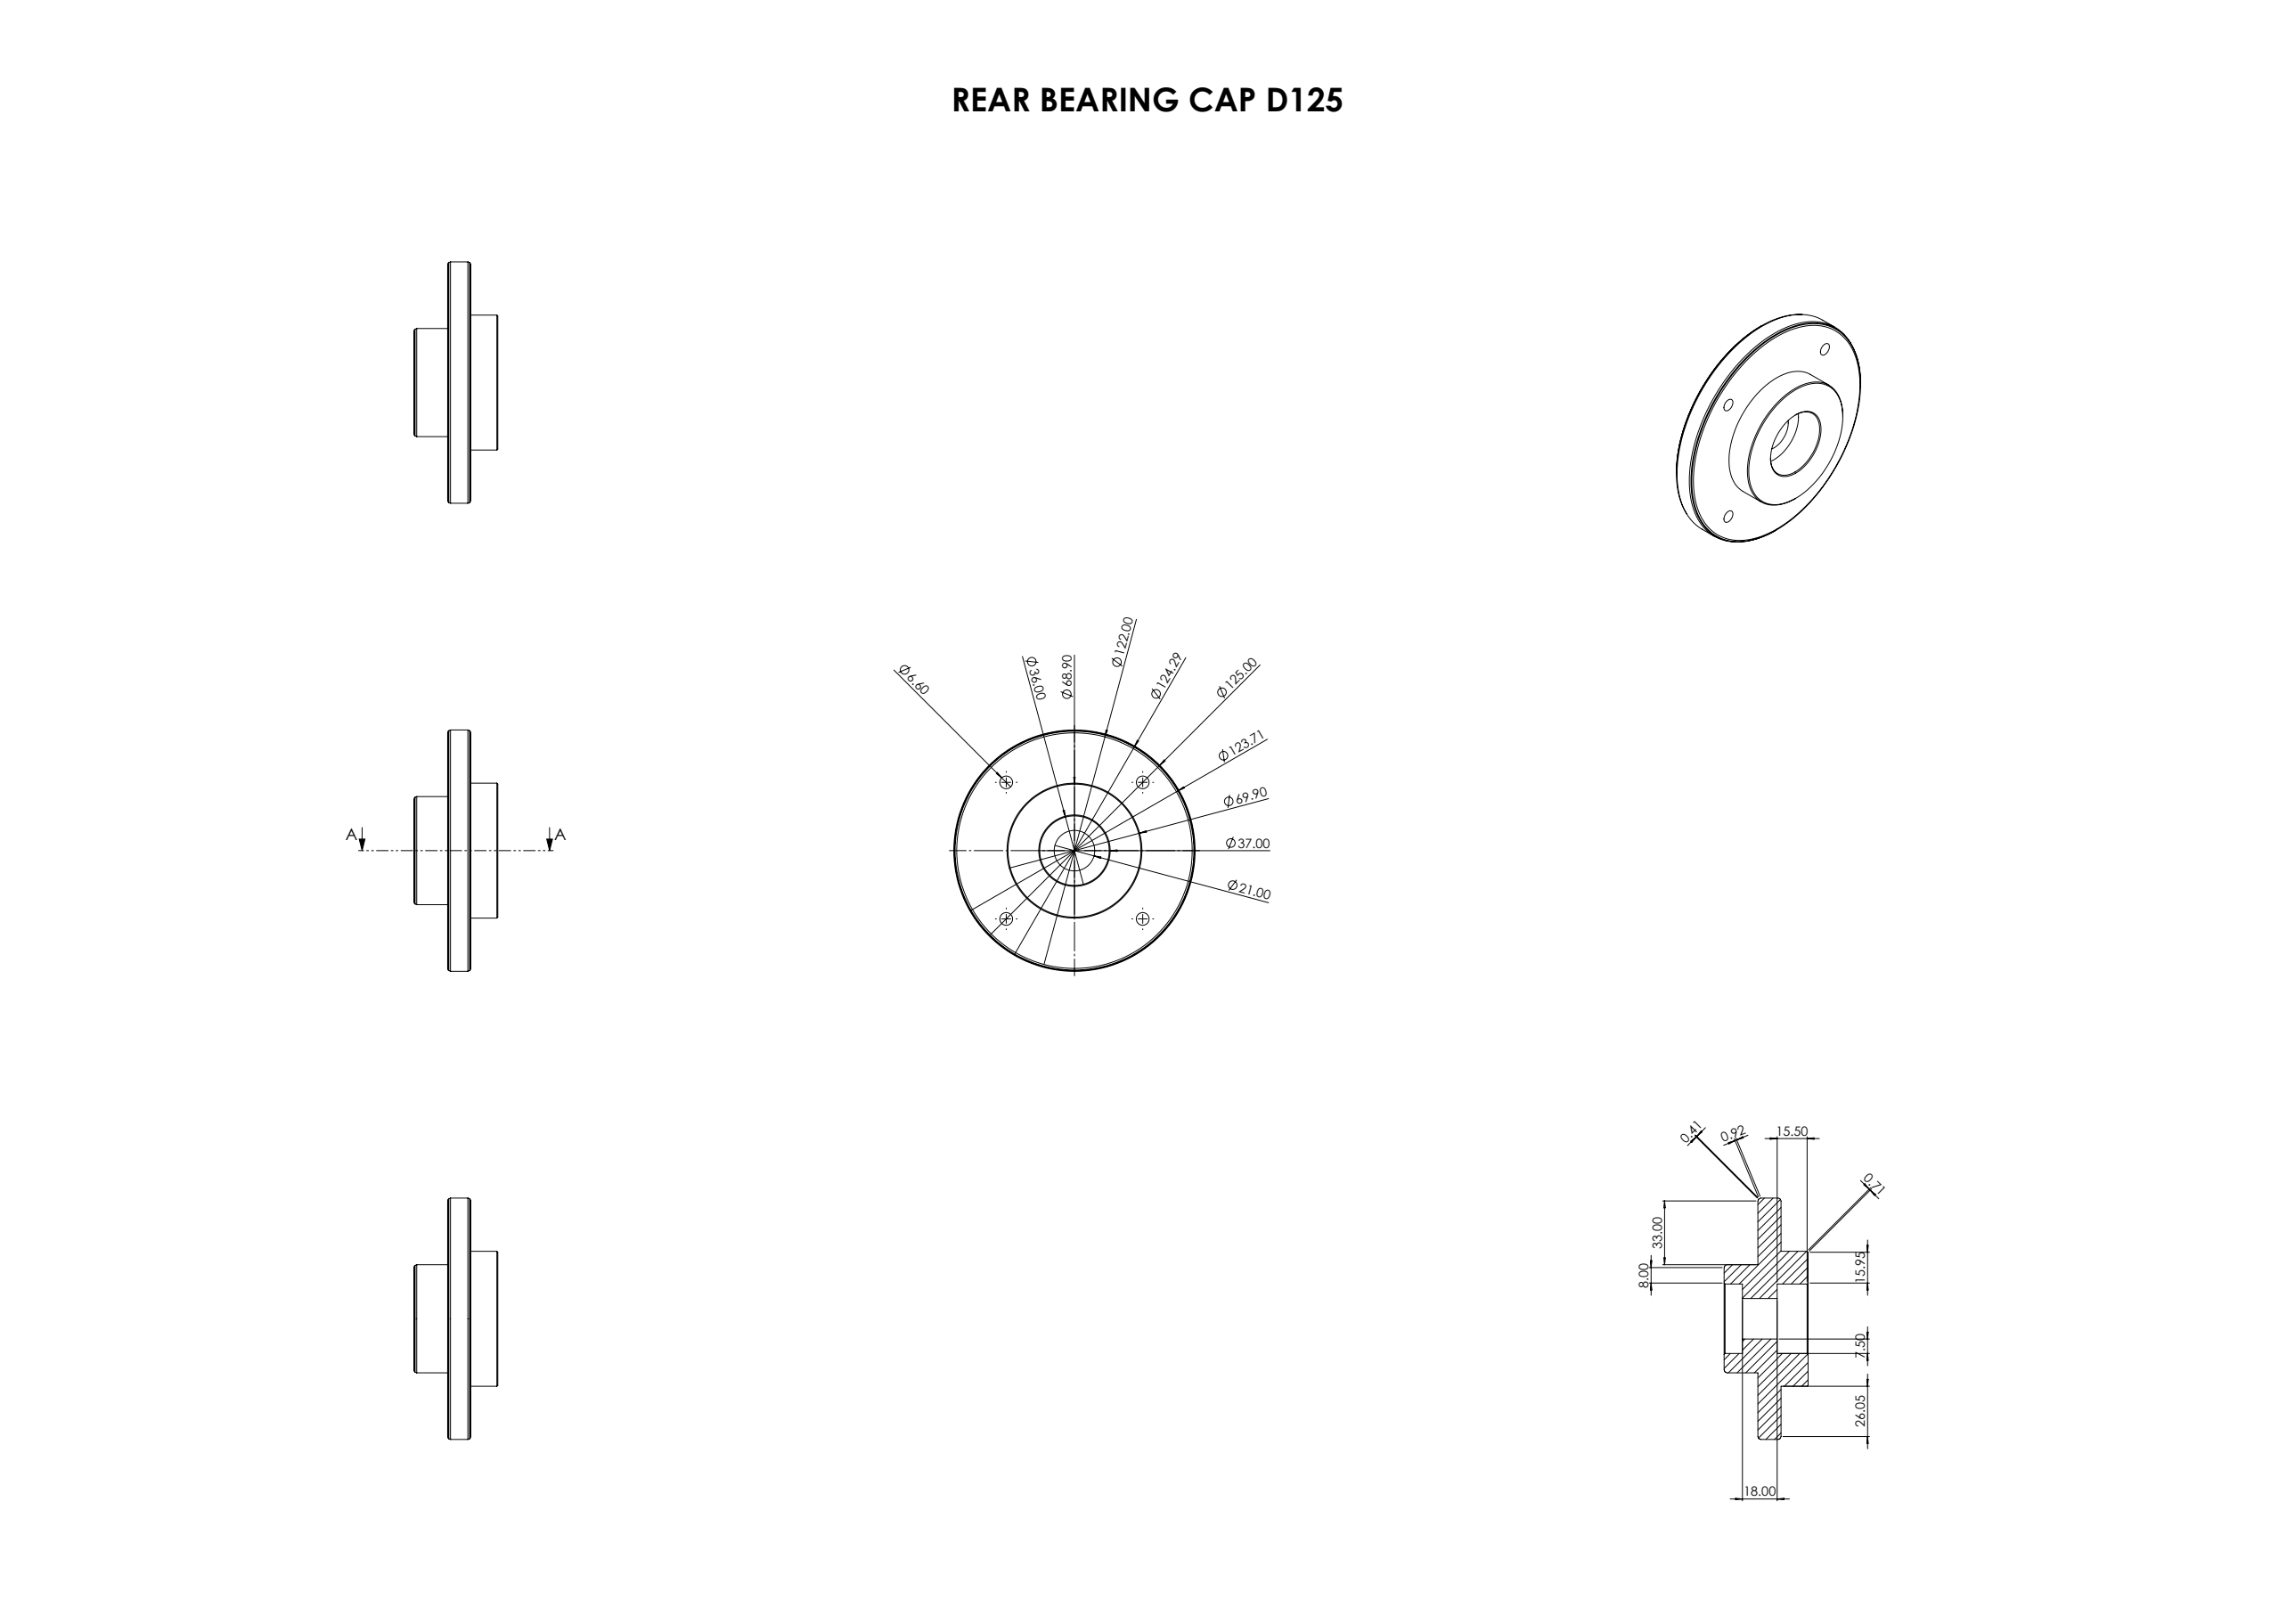
ISO-10303-21;
HEADER;
/* Generated by software containing ST-Developer
 * from STEP Tools, Inc. (www.steptools.com) 
 */

FILE_DESCRIPTION(
/* description */ (''),
/* implementation_level */ '2;1');

FILE_NAME(
/* name */ '07_Rear_Bearing_Cap_D125.step',
/* time_stamp */ '2026-10-26T03:50:32-07:00',
/* author */ (''),
/* organization */ (''),
/* preprocessor_version */ 'ST-DEVELOPER v20.2',
/* originating_system */ 'Autodesk Translation Framework v15.15.0.0',
/* authorisation */ '');

FILE_SCHEMA (('AUTOMOTIVE_DESIGN { 1 0 10303 214 3 1 1 }'));
ENDSEC;

DATA;
#10=MECHANICAL_DESIGN_GEOMETRIC_PRESENTATION_REPRESENTATION('',(#1045),#76660);
#1005=SHAPE_REPRESENTATION_RELATIONSHIP('SRR','None',#76742,#1025);
#1025=ADVANCED_BREP_SHAPE_REPRESENTATION('',(#1065),#76646);
#1045=STYLED_ITEM('',(#76906),#1065);
#1065=MANIFOLD_SOLID_BREP('Rear cap',#26670);
#1255=CYLINDRICAL_SURFACE('',#27760,1.8);
#1256=CYLINDRICAL_SURFACE('',#27778,6.25);
#1257=CYLINDRICAL_SURFACE('',#27803,2.8);
#1258=CYLINDRICAL_SURFACE('',#27811,1.8);
#1259=CYLINDRICAL_SURFACE('',#27813,0.330000000000002);
#1260=CYLINDRICAL_SURFACE('',#27814,0.330000000000002);
#1261=CYLINDRICAL_SURFACE('',#27815,0.330000000000002);
#1262=CYLINDRICAL_SURFACE('',#27816,0.330000000000002);
#1263=CYLINDRICAL_SURFACE('',#27817,3.495);
#1264=CYLINDRICAL_SURFACE('',#27822,1.05);
#1614=FACE_BOUND('',#4700,.T.);
#1615=FACE_BOUND('',#4705,.T.);
#1616=FACE_BOUND('',#4706,.T.);
#1617=FACE_BOUND('',#4707,.T.);
#1618=FACE_BOUND('',#4708,.T.);
#1619=FACE_BOUND('',#4709,.T.);
#1620=FACE_BOUND('',#4716,.T.);
#1621=FACE_BOUND('',#4717,.T.);
#1622=FACE_BOUND('',#4718,.T.);
#1623=FACE_BOUND('',#4719,.T.);
#1624=FACE_BOUND('',#4720,.T.);
#1625=FACE_BOUND('',#4726,.T.);
#1626=FACE_BOUND('',#4736,.T.);
#1627=FACE_BOUND('',#4739,.T.);
#1929=PLANE('',#27758);
#1930=PLANE('',#27769);
#1931=PLANE('',#27789);
#1932=PLANE('',#27806);
#1933=PLANE('',#27820);
#1934=PLANE('',#27824);
#3085=FACE_OUTER_BOUND('',#4698,.T.);
#3086=FACE_OUTER_BOUND('',#4699,.T.);
#3087=FACE_OUTER_BOUND('',#4701,.T.);
#3088=FACE_OUTER_BOUND('',#4702,.T.);
#3089=FACE_OUTER_BOUND('',#4703,.T.);
#3090=FACE_OUTER_BOUND('',#4704,.T.);
#3091=FACE_OUTER_BOUND('',#4710,.T.);
#3092=FACE_OUTER_BOUND('',#4711,.T.);
#3093=FACE_OUTER_BOUND('',#4712,.T.);
#3094=FACE_OUTER_BOUND('',#4713,.T.);
#3095=FACE_OUTER_BOUND('',#4714,.T.);
#3096=FACE_OUTER_BOUND('',#4715,.T.);
#3097=FACE_OUTER_BOUND('',#4721,.T.);
#3098=FACE_OUTER_BOUND('',#4722,.T.);
#3099=FACE_OUTER_BOUND('',#4723,.T.);
#3100=FACE_OUTER_BOUND('',#4724,.T.);
#3101=FACE_OUTER_BOUND('',#4725,.T.);
#3102=FACE_OUTER_BOUND('',#4727,.T.);
#3103=FACE_OUTER_BOUND('',#4728,.T.);
#3104=FACE_OUTER_BOUND('',#4729,.T.);
#3105=FACE_OUTER_BOUND('',#4730,.T.);
#3106=FACE_OUTER_BOUND('',#4731,.T.);
#3107=FACE_OUTER_BOUND('',#4732,.T.);
#3108=FACE_OUTER_BOUND('',#4733,.T.);
#3109=FACE_OUTER_BOUND('',#4734,.T.);
#3110=FACE_OUTER_BOUND('',#4735,.T.);
#3111=FACE_OUTER_BOUND('',#4737,.T.);
#3112=FACE_OUTER_BOUND('',#4738,.T.);
#4698=EDGE_LOOP('',(#19913,#19914,#19915,#19916,#19917));
#4699=EDGE_LOOP('',(#19918));
#4700=EDGE_LOOP('',(#19919));
#4701=EDGE_LOOP('',(#19920,#19921,#19922,#19923,#19924));
#4702=EDGE_LOOP('',(#19925,#19926,#19927,#19928,#19929));
#4703=EDGE_LOOP('',(#19930,#19931,#19932,#19933,#19934,#19935));
#4704=EDGE_LOOP('',(#19936));
#4705=EDGE_LOOP('',(#19937));
#4706=EDGE_LOOP('',(#19938));
#4707=EDGE_LOOP('',(#19939));
#4708=EDGE_LOOP('',(#19940));
#4709=EDGE_LOOP('',(#19941));
#4710=EDGE_LOOP('',(#19942,#19943,#19944,#19945,#19946,#19947));
#4711=EDGE_LOOP('',(#19948,#19949,#19950,#19951,#19952,#19953));
#4712=EDGE_LOOP('',(#19954,#19955,#19956,#19957,#19958,#19959));
#4713=EDGE_LOOP('',(#19960,#19961,#19962,#19963,#19964,#19965));
#4714=EDGE_LOOP('',(#19966,#19967,#19968,#19969,#19970));
#4715=EDGE_LOOP('',(#19971));
#4716=EDGE_LOOP('',(#19972));
#4717=EDGE_LOOP('',(#19973));
#4718=EDGE_LOOP('',(#19974));
#4719=EDGE_LOOP('',(#19975));
#4720=EDGE_LOOP('',(#19976));
#4721=EDGE_LOOP('',(#19977,#19978,#19979,#19980,#19981,#19982));
#4722=EDGE_LOOP('',(#19983,#19984,#19985,#19986,#19987,#19988));
#4723=EDGE_LOOP('',(#19989,#19990,#19991,#19992,#19993));
#4724=EDGE_LOOP('',(#19994,#19995,#19996,#19997,#19998));
#4725=EDGE_LOOP('',(#19999));
#4726=EDGE_LOOP('',(#20000));
#4727=EDGE_LOOP('',(#20001,#20002,#20003,#20004,#20005));
#4728=EDGE_LOOP('',(#20006,#20007,#20008,#20009,#20010));
#4729=EDGE_LOOP('',(#20011,#20012,#20013,#20014));
#4730=EDGE_LOOP('',(#20015,#20016,#20017,#20018));
#4731=EDGE_LOOP('',(#20019,#20020,#20021,#20022));
#4732=EDGE_LOOP('',(#20023,#20024,#20025,#20026));
#4733=EDGE_LOOP('',(#20027,#20028,#20029,#20030));
#4734=EDGE_LOOP('',(#20031,#20032,#20033,#20034));
#4735=EDGE_LOOP('',(#20035));
#4736=EDGE_LOOP('',(#20036));
#4737=EDGE_LOOP('',(#20037,#20038,#20039,#20040));
#4738=EDGE_LOOP('',(#20041));
#4739=EDGE_LOOP('',(#20042));
#6023=CIRCLE('',#27755,1.8);
#6024=CIRCLE('',#27756,1.8);
#6025=CIRCLE('',#27757,1.85);
#6026=CIRCLE('',#27759,3.445);
#6027=CIRCLE('',#27761,1.8);
#6028=CIRCLE('',#27763,6.1);
#6029=CIRCLE('',#27764,6.18535533905933);
#6030=CIRCLE('',#27765,6.18535533905933);
#6031=CIRCLE('',#27767,6.21464466094067);
#6032=CIRCLE('',#27768,6.21464466094067);
#6033=CIRCLE('',#27770,3.495);
#6034=CIRCLE('',#27771,0.330000000000002);
#6035=CIRCLE('',#27772,0.330000000000002);
#6036=CIRCLE('',#27773,0.330000000000002);
#6037=CIRCLE('',#27774,0.330000000000002);
#6038=CIRCLE('',#27776,6.25);
#6039=CIRCLE('',#27777,6.25);
#6040=CIRCLE('',#27779,6.25);
#6041=CIRCLE('',#27780,6.25);
#6042=CIRCLE('',#27782,6.21464466094067);
#6043=CIRCLE('',#27783,6.21464466094067);
#6044=CIRCLE('',#27785,6.18535533905933);
#6045=CIRCLE('',#27786,6.18535533905933);
#6046=CIRCLE('',#27788,6.1);
#6047=CIRCLE('',#27790,2.8);
#6048=CIRCLE('',#27791,0.330000000000002);
#6049=CIRCLE('',#27792,0.330000000000002);
#6050=CIRCLE('',#27793,0.330000000000002);
#6051=CIRCLE('',#27794,0.330000000000002);
#6052=CIRCLE('',#27796,2.8);
#6053=CIRCLE('',#27797,2.8);
#6054=CIRCLE('',#27798,2.76464466094067);
#6055=CIRCLE('',#27799,2.76464466094067);
#6056=CIRCLE('',#27801,2.73535533905933);
#6057=CIRCLE('',#27802,2.73535533905933);
#6058=CIRCLE('',#27805,2.65);
#6059=CIRCLE('',#27807,1.85);
#6060=CIRCLE('',#27809,1.8);
#6061=CIRCLE('',#27810,1.8);
#6062=CIRCLE('',#27812,1.8);
#6063=CIRCLE('',#27818,3.495);
#6064=CIRCLE('',#27821,1.05);
#6065=CIRCLE('',#27823,1.05);
#7407=LINE('',#49695,#9563);
#7408=LINE('',#49702,#9564);
#7409=LINE('',#49708,#9565);
#7410=LINE('',#49714,#9566);
#7411=LINE('',#49731,#9567);
#7412=LINE('',#49737,#9568);
#7413=LINE('',#49743,#9569);
#7414=LINE('',#49749,#9570);
#7415=LINE('',#49755,#9571);
#7416=LINE('',#49774,#9572);
#7417=LINE('',#49780,#9573);
#7418=LINE('',#49785,#9574);
#7419=LINE('',#49788,#9575);
#7420=LINE('',#49795,#9576);
#7421=LINE('',#49802,#9577);
#7422=LINE('',#49804,#9578);
#7423=LINE('',#49806,#9579);
#7424=LINE('',#49808,#9580);
#7425=LINE('',#49810,#9581);
#7426=LINE('',#49814,#9582);
#7427=LINE('',#49816,#9583);
#7428=LINE('',#49822,#9584);
#9563=VECTOR('',#31864,1.825);
#9564=VECTOR('',#31873,1.8);
#9565=VECTOR('',#31880,6.14267766952966);
#9566=VECTOR('',#31887,6.2);
#9567=VECTOR('',#31906,6.23232233047034);
#9568=VECTOR('',#31913,6.25);
#9569=VECTOR('',#31920,6.23232233047034);
#9570=VECTOR('',#31927,6.2);
#9571=VECTOR('',#31934,6.14267766952966);
#9572=VECTOR('',#31955,2.78232233047034);
#9573=VECTOR('',#31962,2.75);
#9574=VECTOR('',#31969,2.8);
#9575=VECTOR('',#31972,2.69267766952966);
#9576=VECTOR('',#31981,1.825);
#9577=VECTOR('',#31990,1.8);
#9578=VECTOR('',#31993,0.330000000000002);
#9579=VECTOR('',#31996,0.330000000000002);
#9580=VECTOR('',#31999,0.330000000000002);
#9581=VECTOR('',#32002,0.330000000000002);
#9582=VECTOR('',#32007,3.495);
#9583=VECTOR('',#32010,3.47);
#9584=VECTOR('',#32017,1.05);
#11754=VERTEX_POINT('',#49690);
#11755=VERTEX_POINT('',#49691);
#11756=VERTEX_POINT('',#49694);
#11757=VERTEX_POINT('',#49698);
#11758=VERTEX_POINT('',#49701);
#11759=VERTEX_POINT('',#49705);
#11760=VERTEX_POINT('',#49707);
#11761=VERTEX_POINT('',#49709);
#11762=VERTEX_POINT('',#49713);
#11763=VERTEX_POINT('',#49715);
#11764=VERTEX_POINT('',#49719);
#11765=VERTEX_POINT('',#49721);
#11766=VERTEX_POINT('',#49723);
#11767=VERTEX_POINT('',#49725);
#11768=VERTEX_POINT('',#49727);
#11769=VERTEX_POINT('',#49730);
#11770=VERTEX_POINT('',#49732);
#11771=VERTEX_POINT('',#49736);
#11772=VERTEX_POINT('',#49738);
#11773=VERTEX_POINT('',#49742);
#11774=VERTEX_POINT('',#49744);
#11775=VERTEX_POINT('',#49748);
#11776=VERTEX_POINT('',#49750);
#11777=VERTEX_POINT('',#49754);
#11778=VERTEX_POINT('',#49758);
#11779=VERTEX_POINT('',#49760);
#11780=VERTEX_POINT('',#49762);
#11781=VERTEX_POINT('',#49764);
#11782=VERTEX_POINT('',#49766);
#11783=VERTEX_POINT('',#49769);
#11784=VERTEX_POINT('',#49770);
#11785=VERTEX_POINT('',#49773);
#11786=VERTEX_POINT('',#49775);
#11787=VERTEX_POINT('',#49779);
#11788=VERTEX_POINT('',#49781);
#11789=VERTEX_POINT('',#49787);
#11790=VERTEX_POINT('',#49791);
#11791=VERTEX_POINT('',#49794);
#11792=VERTEX_POINT('',#49796);
#11793=VERTEX_POINT('',#49800);
#11794=VERTEX_POINT('',#49812);
#11795=VERTEX_POINT('',#49818);
#11796=VERTEX_POINT('',#49821);
#14679=EDGE_CURVE('',#11754,#11755,#6023,.T.);
#14680=EDGE_CURVE('',#11755,#11754,#6024,.T.);
#14681=EDGE_CURVE('',#11754,#11756,#7407,.T.);
#14682=EDGE_CURVE('',#11756,#11756,#6025,.T.);
#14683=EDGE_CURVE('',#11757,#11757,#6026,.T.);
#14684=EDGE_CURVE('',#11755,#11758,#7408,.T.);
#14685=EDGE_CURVE('',#11758,#11758,#6027,.T.);
#14686=EDGE_CURVE('',#11759,#11759,#6028,.T.);
#14687=EDGE_CURVE('',#11759,#11760,#7409,.T.);
#14688=EDGE_CURVE('',#11760,#11761,#6029,.T.);
#14689=EDGE_CURVE('',#11761,#11760,#6030,.T.);
#14690=EDGE_CURVE('',#11761,#11762,#7410,.T.);
#14691=EDGE_CURVE('',#11763,#11762,#6031,.T.);
#14692=EDGE_CURVE('',#11762,#11763,#6032,.T.);
#14693=EDGE_CURVE('',#11764,#11764,#6033,.T.);
#14694=EDGE_CURVE('',#11765,#11765,#6034,.T.);
#14695=EDGE_CURVE('',#11766,#11766,#6035,.T.);
#14696=EDGE_CURVE('',#11767,#11767,#6036,.T.);
#14697=EDGE_CURVE('',#11768,#11768,#6037,.T.);
#14698=EDGE_CURVE('',#11763,#11769,#7411,.T.);
#14699=EDGE_CURVE('',#11769,#11770,#6038,.T.);
#14700=EDGE_CURVE('',#11770,#11769,#6039,.T.);
#14701=EDGE_CURVE('',#11770,#11771,#7412,.T.);
#14702=EDGE_CURVE('',#11772,#11771,#6040,.T.);
#14703=EDGE_CURVE('',#11771,#11772,#6041,.T.);
#14704=EDGE_CURVE('',#11772,#11773,#7413,.T.);
#14705=EDGE_CURVE('',#11773,#11774,#6042,.T.);
#14706=EDGE_CURVE('',#11774,#11773,#6043,.T.);
#14707=EDGE_CURVE('',#11774,#11775,#7414,.T.);
#14708=EDGE_CURVE('',#11776,#11775,#6044,.T.);
#14709=EDGE_CURVE('',#11775,#11776,#6045,.T.);
#14710=EDGE_CURVE('',#11776,#11777,#7415,.T.);
#14711=EDGE_CURVE('',#11777,#11777,#6046,.T.);
#14712=EDGE_CURVE('',#11778,#11778,#6047,.T.);
#14713=EDGE_CURVE('',#11779,#11779,#6048,.T.);
#14714=EDGE_CURVE('',#11780,#11780,#6049,.T.);
#14715=EDGE_CURVE('',#11781,#11781,#6050,.T.);
#14716=EDGE_CURVE('',#11782,#11782,#6051,.T.);
#14717=EDGE_CURVE('',#11783,#11784,#6052,.T.);
#14718=EDGE_CURVE('',#11784,#11783,#6053,.T.);
#14719=EDGE_CURVE('',#11783,#11785,#7416,.T.);
#14720=EDGE_CURVE('',#11785,#11786,#6054,.T.);
#14721=EDGE_CURVE('',#11786,#11785,#6055,.T.);
#14722=EDGE_CURVE('',#11786,#11787,#7417,.T.);
#14723=EDGE_CURVE('',#11788,#11787,#6056,.T.);
#14724=EDGE_CURVE('',#11787,#11788,#6057,.T.);
#14725=EDGE_CURVE('',#11778,#11784,#7418,.T.);
#14726=EDGE_CURVE('',#11788,#11789,#7419,.T.);
#14727=EDGE_CURVE('',#11789,#11789,#6058,.T.);
#14728=EDGE_CURVE('',#11790,#11790,#6059,.T.);
#14729=EDGE_CURVE('',#11790,#11791,#7420,.T.);
#14730=EDGE_CURVE('',#11791,#11792,#6060,.T.);
#14731=EDGE_CURVE('',#11792,#11791,#6061,.T.);
#14732=EDGE_CURVE('',#11793,#11793,#6062,.T.);
#14733=EDGE_CURVE('',#11793,#11792,#7421,.T.);
#14734=EDGE_CURVE('',#11768,#11782,#7422,.T.);
#14735=EDGE_CURVE('',#11767,#11781,#7423,.T.);
#14736=EDGE_CURVE('',#11766,#11780,#7424,.T.);
#14737=EDGE_CURVE('',#11765,#11779,#7425,.T.);
#14738=EDGE_CURVE('',#11794,#11794,#6063,.T.);
#14739=EDGE_CURVE('',#11794,#11764,#7426,.T.);
#14740=EDGE_CURVE('',#11757,#11794,#7427,.T.);
#14741=EDGE_CURVE('',#11795,#11795,#6064,.T.);
#14742=EDGE_CURVE('',#11795,#11796,#7428,.T.);
#14743=EDGE_CURVE('',#11796,#11796,#6065,.T.);
#19913=ORIENTED_EDGE('',*,*,#14679,.T.);
#19914=ORIENTED_EDGE('',*,*,#14680,.T.);
#19915=ORIENTED_EDGE('',*,*,#14681,.T.);
#19916=ORIENTED_EDGE('',*,*,#14682,.T.);
#19917=ORIENTED_EDGE('',*,*,#14681,.F.);
#19918=ORIENTED_EDGE('',*,*,#14683,.T.);
#19919=ORIENTED_EDGE('',*,*,#14682,.F.);
#19920=ORIENTED_EDGE('',*,*,#14679,.F.);
#19921=ORIENTED_EDGE('',*,*,#14680,.F.);
#19922=ORIENTED_EDGE('',*,*,#14684,.T.);
#19923=ORIENTED_EDGE('',*,*,#14685,.F.);
#19924=ORIENTED_EDGE('',*,*,#14684,.F.);
#19925=ORIENTED_EDGE('',*,*,#14686,.T.);
#19926=ORIENTED_EDGE('',*,*,#14687,.T.);
#19927=ORIENTED_EDGE('',*,*,#14688,.T.);
#19928=ORIENTED_EDGE('',*,*,#14689,.T.);
#19929=ORIENTED_EDGE('',*,*,#14687,.F.);
#19930=ORIENTED_EDGE('',*,*,#14688,.F.);
#19931=ORIENTED_EDGE('',*,*,#14689,.F.);
#19932=ORIENTED_EDGE('',*,*,#14690,.T.);
#19933=ORIENTED_EDGE('',*,*,#14691,.F.);
#19934=ORIENTED_EDGE('',*,*,#14692,.F.);
#19935=ORIENTED_EDGE('',*,*,#14690,.F.);
#19936=ORIENTED_EDGE('',*,*,#14686,.F.);
#19937=ORIENTED_EDGE('',*,*,#14693,.F.);
#19938=ORIENTED_EDGE('',*,*,#14694,.T.);
#19939=ORIENTED_EDGE('',*,*,#14695,.T.);
#19940=ORIENTED_EDGE('',*,*,#14696,.T.);
#19941=ORIENTED_EDGE('',*,*,#14697,.T.);
#19942=ORIENTED_EDGE('',*,*,#14691,.T.);
#19943=ORIENTED_EDGE('',*,*,#14692,.T.);
#19944=ORIENTED_EDGE('',*,*,#14698,.T.);
#19945=ORIENTED_EDGE('',*,*,#14699,.T.);
#19946=ORIENTED_EDGE('',*,*,#14700,.T.);
#19947=ORIENTED_EDGE('',*,*,#14698,.F.);
#19948=ORIENTED_EDGE('',*,*,#14699,.F.);
#19949=ORIENTED_EDGE('',*,*,#14700,.F.);
#19950=ORIENTED_EDGE('',*,*,#14701,.T.);
#19951=ORIENTED_EDGE('',*,*,#14702,.F.);
#19952=ORIENTED_EDGE('',*,*,#14703,.F.);
#19953=ORIENTED_EDGE('',*,*,#14701,.F.);
#19954=ORIENTED_EDGE('',*,*,#14702,.T.);
#19955=ORIENTED_EDGE('',*,*,#14703,.T.);
#19956=ORIENTED_EDGE('',*,*,#14704,.T.);
#19957=ORIENTED_EDGE('',*,*,#14705,.T.);
#19958=ORIENTED_EDGE('',*,*,#14706,.T.);
#19959=ORIENTED_EDGE('',*,*,#14704,.F.);
#19960=ORIENTED_EDGE('',*,*,#14705,.F.);
#19961=ORIENTED_EDGE('',*,*,#14706,.F.);
#19962=ORIENTED_EDGE('',*,*,#14707,.T.);
#19963=ORIENTED_EDGE('',*,*,#14708,.F.);
#19964=ORIENTED_EDGE('',*,*,#14709,.F.);
#19965=ORIENTED_EDGE('',*,*,#14707,.F.);
#19966=ORIENTED_EDGE('',*,*,#14708,.T.);
#19967=ORIENTED_EDGE('',*,*,#14709,.T.);
#19968=ORIENTED_EDGE('',*,*,#14710,.T.);
#19969=ORIENTED_EDGE('',*,*,#14711,.T.);
#19970=ORIENTED_EDGE('',*,*,#14710,.F.);
#19971=ORIENTED_EDGE('',*,*,#14711,.F.);
#19972=ORIENTED_EDGE('',*,*,#14712,.T.);
#19973=ORIENTED_EDGE('',*,*,#14713,.T.);
#19974=ORIENTED_EDGE('',*,*,#14714,.T.);
#19975=ORIENTED_EDGE('',*,*,#14715,.T.);
#19976=ORIENTED_EDGE('',*,*,#14716,.T.);
#19977=ORIENTED_EDGE('',*,*,#14717,.T.);
#19978=ORIENTED_EDGE('',*,*,#14718,.T.);
#19979=ORIENTED_EDGE('',*,*,#14719,.T.);
#19980=ORIENTED_EDGE('',*,*,#14720,.T.);
#19981=ORIENTED_EDGE('',*,*,#14721,.T.);
#19982=ORIENTED_EDGE('',*,*,#14719,.F.);
#19983=ORIENTED_EDGE('',*,*,#14720,.F.);
#19984=ORIENTED_EDGE('',*,*,#14721,.F.);
#19985=ORIENTED_EDGE('',*,*,#14722,.T.);
#19986=ORIENTED_EDGE('',*,*,#14723,.F.);
#19987=ORIENTED_EDGE('',*,*,#14724,.F.);
#19988=ORIENTED_EDGE('',*,*,#14722,.F.);
#19989=ORIENTED_EDGE('',*,*,#14712,.F.);
#19990=ORIENTED_EDGE('',*,*,#14725,.T.);
#19991=ORIENTED_EDGE('',*,*,#14717,.F.);
#19992=ORIENTED_EDGE('',*,*,#14718,.F.);
#19993=ORIENTED_EDGE('',*,*,#14725,.F.);
#19994=ORIENTED_EDGE('',*,*,#14723,.T.);
#19995=ORIENTED_EDGE('',*,*,#14724,.T.);
#19996=ORIENTED_EDGE('',*,*,#14726,.T.);
#19997=ORIENTED_EDGE('',*,*,#14727,.T.);
#19998=ORIENTED_EDGE('',*,*,#14726,.F.);
#19999=ORIENTED_EDGE('',*,*,#14727,.F.);
#20000=ORIENTED_EDGE('',*,*,#14728,.F.);
#20001=ORIENTED_EDGE('',*,*,#14728,.T.);
#20002=ORIENTED_EDGE('',*,*,#14729,.T.);
#20003=ORIENTED_EDGE('',*,*,#14730,.T.);
#20004=ORIENTED_EDGE('',*,*,#14731,.T.);
#20005=ORIENTED_EDGE('',*,*,#14729,.F.);
#20006=ORIENTED_EDGE('',*,*,#14732,.T.);
#20007=ORIENTED_EDGE('',*,*,#14733,.T.);
#20008=ORIENTED_EDGE('',*,*,#14730,.F.);
#20009=ORIENTED_EDGE('',*,*,#14731,.F.);
#20010=ORIENTED_EDGE('',*,*,#14733,.F.);
#20011=ORIENTED_EDGE('',*,*,#14697,.F.);
#20012=ORIENTED_EDGE('',*,*,#14734,.T.);
#20013=ORIENTED_EDGE('',*,*,#14716,.F.);
#20014=ORIENTED_EDGE('',*,*,#14734,.F.);
#20015=ORIENTED_EDGE('',*,*,#14696,.F.);
#20016=ORIENTED_EDGE('',*,*,#14735,.T.);
#20017=ORIENTED_EDGE('',*,*,#14715,.F.);
#20018=ORIENTED_EDGE('',*,*,#14735,.F.);
#20019=ORIENTED_EDGE('',*,*,#14695,.F.);
#20020=ORIENTED_EDGE('',*,*,#14736,.T.);
#20021=ORIENTED_EDGE('',*,*,#14714,.F.);
#20022=ORIENTED_EDGE('',*,*,#14736,.F.);
#20023=ORIENTED_EDGE('',*,*,#14694,.F.);
#20024=ORIENTED_EDGE('',*,*,#14737,.T.);
#20025=ORIENTED_EDGE('',*,*,#14713,.F.);
#20026=ORIENTED_EDGE('',*,*,#14737,.F.);
#20027=ORIENTED_EDGE('',*,*,#14738,.F.);
#20028=ORIENTED_EDGE('',*,*,#14739,.T.);
#20029=ORIENTED_EDGE('',*,*,#14693,.T.);
#20030=ORIENTED_EDGE('',*,*,#14739,.F.);
#20031=ORIENTED_EDGE('',*,*,#14683,.F.);
#20032=ORIENTED_EDGE('',*,*,#14740,.T.);
#20033=ORIENTED_EDGE('',*,*,#14738,.T.);
#20034=ORIENTED_EDGE('',*,*,#14740,.F.);
#20035=ORIENTED_EDGE('',*,*,#14685,.T.);
#20036=ORIENTED_EDGE('',*,*,#14741,.F.);
#20037=ORIENTED_EDGE('',*,*,#14741,.T.);
#20038=ORIENTED_EDGE('',*,*,#14742,.T.);
#20039=ORIENTED_EDGE('',*,*,#14743,.F.);
#20040=ORIENTED_EDGE('',*,*,#14742,.F.);
#20041=ORIENTED_EDGE('',*,*,#14732,.F.);
#20042=ORIENTED_EDGE('',*,*,#14743,.T.);
#25033=CONICAL_SURFACE('',#27754,1.825,0.785398163397442);
#25034=CONICAL_SURFACE('',#27762,6.14267766952966,1.17809724509617);
#25035=CONICAL_SURFACE('',#27766,6.2,0.785398163397448);
#25036=CONICAL_SURFACE('',#27775,6.23232233047034,0.392699081698724);
#25037=CONICAL_SURFACE('',#27781,6.23232233047034,0.392699081698724);
#25038=CONICAL_SURFACE('',#27784,6.2,0.785398163397444);
#25039=CONICAL_SURFACE('',#27787,6.14267766952966,1.17809724509617);
#25040=CONICAL_SURFACE('',#27795,2.78232233047034,0.39269908169872);
#25041=CONICAL_SURFACE('',#27800,2.75,0.785398163397444);
#25042=CONICAL_SURFACE('',#27804,2.69267766952966,1.17809724509617);
#25043=CONICAL_SURFACE('',#27808,1.825,0.785398163397451);
#25044=CONICAL_SURFACE('',#27819,3.47,0.785398163397439);
#25673=ADVANCED_FACE('',(#3085),#25033,.F.);
#25674=ADVANCED_FACE('',(#3086,#1614),#1929,.T.);
#25675=ADVANCED_FACE('',(#3087),#1255,.F.);
#25676=ADVANCED_FACE('',(#3088),#25034,.T.);
#25677=ADVANCED_FACE('',(#3089),#25035,.T.);
#25678=ADVANCED_FACE('',(#3090,#1615,#1616,#1617,#1618,#1619),#1930,.T.);
#25679=ADVANCED_FACE('',(#3091),#25036,.T.);
#25680=ADVANCED_FACE('',(#3092),#1256,.T.);
#25681=ADVANCED_FACE('',(#3093),#25037,.T.);
#25682=ADVANCED_FACE('',(#3094),#25038,.T.);
#25683=ADVANCED_FACE('',(#3095),#25039,.T.);
#25684=ADVANCED_FACE('',(#3096,#1620,#1621,#1622,#1623,#1624),#1931,.T.);
#25685=ADVANCED_FACE('',(#3097),#25040,.T.);
#25686=ADVANCED_FACE('',(#3098),#25041,.T.);
#25687=ADVANCED_FACE('',(#3099),#1257,.T.);
#25688=ADVANCED_FACE('',(#3100),#25042,.T.);
#25689=ADVANCED_FACE('',(#3101,#1625),#1932,.T.);
#25690=ADVANCED_FACE('',(#3102),#25043,.F.);
#25691=ADVANCED_FACE('',(#3103),#1258,.F.);
#25692=ADVANCED_FACE('',(#3104),#1259,.F.);
#25693=ADVANCED_FACE('',(#3105),#1260,.F.);
#25694=ADVANCED_FACE('',(#3106),#1261,.F.);
#25695=ADVANCED_FACE('',(#3107),#1262,.F.);
#25696=ADVANCED_FACE('',(#3108),#1263,.T.);
#25697=ADVANCED_FACE('',(#3109),#25044,.T.);
#25698=ADVANCED_FACE('',(#3110,#1626),#1933,.T.);
#25699=ADVANCED_FACE('',(#3111),#1264,.F.);
#25700=ADVANCED_FACE('',(#3112,#1627),#1934,.T.);
#26670=CLOSED_SHELL('',(#25673,#25674,#25675,#25676,#25677,#25678,#25679,
#25680,#25681,#25682,#25683,#25684,#25685,#25686,#25687,#25688,#25689,#25690,
#25691,#25692,#25693,#25694,#25695,#25696,#25697,#25698,#25699,#25700));
#27753=AXIS2_PLACEMENT_3D('',#49688,#31856,#31857);
#27754=AXIS2_PLACEMENT_3D('',#49689,#31858,#31859);
#27755=AXIS2_PLACEMENT_3D('',#49692,#31860,#31861);
#27756=AXIS2_PLACEMENT_3D('',#49693,#31862,#31863);
#27757=AXIS2_PLACEMENT_3D('',#49696,#31865,#31866);
#27758=AXIS2_PLACEMENT_3D('',#49697,#31867,#31868);
#27759=AXIS2_PLACEMENT_3D('',#49699,#31869,#31870);
#27760=AXIS2_PLACEMENT_3D('',#49700,#31871,#31872);
#27761=AXIS2_PLACEMENT_3D('',#49703,#31874,#31875);
#27762=AXIS2_PLACEMENT_3D('',#49704,#31876,#31877);
#27763=AXIS2_PLACEMENT_3D('',#49706,#31878,#31879);
#27764=AXIS2_PLACEMENT_3D('',#49710,#31881,#31882);
#27765=AXIS2_PLACEMENT_3D('',#49711,#31883,#31884);
#27766=AXIS2_PLACEMENT_3D('',#49712,#31885,#31886);
#27767=AXIS2_PLACEMENT_3D('',#49716,#31888,#31889);
#27768=AXIS2_PLACEMENT_3D('',#49717,#31890,#31891);
#27769=AXIS2_PLACEMENT_3D('',#49718,#31892,#31893);
#27770=AXIS2_PLACEMENT_3D('',#49720,#31894,#31895);
#27771=AXIS2_PLACEMENT_3D('',#49722,#31896,#31897);
#27772=AXIS2_PLACEMENT_3D('',#49724,#31898,#31899);
#27773=AXIS2_PLACEMENT_3D('',#49726,#31900,#31901);
#27774=AXIS2_PLACEMENT_3D('',#49728,#31902,#31903);
#27775=AXIS2_PLACEMENT_3D('',#49729,#31904,#31905);
#27776=AXIS2_PLACEMENT_3D('',#49733,#31907,#31908);
#27777=AXIS2_PLACEMENT_3D('',#49734,#31909,#31910);
#27778=AXIS2_PLACEMENT_3D('',#49735,#31911,#31912);
#27779=AXIS2_PLACEMENT_3D('',#49739,#31914,#31915);
#27780=AXIS2_PLACEMENT_3D('',#49740,#31916,#31917);
#27781=AXIS2_PLACEMENT_3D('',#49741,#31918,#31919);
#27782=AXIS2_PLACEMENT_3D('',#49745,#31921,#31922);
#27783=AXIS2_PLACEMENT_3D('',#49746,#31923,#31924);
#27784=AXIS2_PLACEMENT_3D('',#49747,#31925,#31926);
#27785=AXIS2_PLACEMENT_3D('',#49751,#31928,#31929);
#27786=AXIS2_PLACEMENT_3D('',#49752,#31930,#31931);
#27787=AXIS2_PLACEMENT_3D('',#49753,#31932,#31933);
#27788=AXIS2_PLACEMENT_3D('',#49756,#31935,#31936);
#27789=AXIS2_PLACEMENT_3D('',#49757,#31937,#31938);
#27790=AXIS2_PLACEMENT_3D('',#49759,#31939,#31940);
#27791=AXIS2_PLACEMENT_3D('',#49761,#31941,#31942);
#27792=AXIS2_PLACEMENT_3D('',#49763,#31943,#31944);
#27793=AXIS2_PLACEMENT_3D('',#49765,#31945,#31946);
#27794=AXIS2_PLACEMENT_3D('',#49767,#31947,#31948);
#27795=AXIS2_PLACEMENT_3D('',#49768,#31949,#31950);
#27796=AXIS2_PLACEMENT_3D('',#49771,#31951,#31952);
#27797=AXIS2_PLACEMENT_3D('',#49772,#31953,#31954);
#27798=AXIS2_PLACEMENT_3D('',#49776,#31956,#31957);
#27799=AXIS2_PLACEMENT_3D('',#49777,#31958,#31959);
#27800=AXIS2_PLACEMENT_3D('',#49778,#31960,#31961);
#27801=AXIS2_PLACEMENT_3D('',#49782,#31963,#31964);
#27802=AXIS2_PLACEMENT_3D('',#49783,#31965,#31966);
#27803=AXIS2_PLACEMENT_3D('',#49784,#31967,#31968);
#27804=AXIS2_PLACEMENT_3D('',#49786,#31970,#31971);
#27805=AXIS2_PLACEMENT_3D('',#49789,#31973,#31974);
#27806=AXIS2_PLACEMENT_3D('',#49790,#31975,#31976);
#27807=AXIS2_PLACEMENT_3D('',#49792,#31977,#31978);
#27808=AXIS2_PLACEMENT_3D('',#49793,#31979,#31980);
#27809=AXIS2_PLACEMENT_3D('',#49797,#31982,#31983);
#27810=AXIS2_PLACEMENT_3D('',#49798,#31984,#31985);
#27811=AXIS2_PLACEMENT_3D('',#49799,#31986,#31987);
#27812=AXIS2_PLACEMENT_3D('',#49801,#31988,#31989);
#27813=AXIS2_PLACEMENT_3D('',#49803,#31991,#31992);
#27814=AXIS2_PLACEMENT_3D('',#49805,#31994,#31995);
#27815=AXIS2_PLACEMENT_3D('',#49807,#31997,#31998);
#27816=AXIS2_PLACEMENT_3D('',#49809,#32000,#32001);
#27817=AXIS2_PLACEMENT_3D('',#49811,#32003,#32004);
#27818=AXIS2_PLACEMENT_3D('',#49813,#32005,#32006);
#27819=AXIS2_PLACEMENT_3D('',#49815,#32008,#32009);
#27820=AXIS2_PLACEMENT_3D('',#49817,#32011,#32012);
#27821=AXIS2_PLACEMENT_3D('',#49819,#32013,#32014);
#27822=AXIS2_PLACEMENT_3D('',#49820,#32015,#32016);
#27823=AXIS2_PLACEMENT_3D('',#49823,#32018,#32019);
#27824=AXIS2_PLACEMENT_3D('',#49824,#32020,#32021);
#31856=DIRECTION('axis',(0.,0.,1.));
#31857=DIRECTION('refdir',(1.,0.,0.));
#31858=DIRECTION('center_axis',(1.,0.,0.));
#31859=DIRECTION('ref_axis',(0.,-1.,0.));
#31860=DIRECTION('center_axis',(-1.,0.,0.));
#31861=DIRECTION('ref_axis',(0.,-1.,0.));
#31862=DIRECTION('center_axis',(-1.,0.,0.));
#31863=DIRECTION('ref_axis',(0.,-1.,0.));
#31864=DIRECTION('',(0.707106781186552,0.707106781186543,-8.65956056235487E-17));
#31865=DIRECTION('center_axis',(1.,0.,0.));
#31866=DIRECTION('ref_axis',(0.,-1.,0.));
#31867=DIRECTION('center_axis',(1.,0.,0.));
#31868=DIRECTION('ref_axis',(0.,0.,-1.));
#31869=DIRECTION('center_axis',(1.,0.,0.));
#31870=DIRECTION('ref_axis',(0.,0.,-1.));
#31871=DIRECTION('center_axis',(1.,0.,0.));
#31872=DIRECTION('ref_axis',(0.,1.,0.));
#31873=DIRECTION('',(-1.,0.,0.));
#31874=DIRECTION('center_axis',(1.,0.,0.));
#31875=DIRECTION('ref_axis',(0.,0.,-1.));
#31876=DIRECTION('center_axis',(-1.,0.,0.));
#31877=DIRECTION('ref_axis',(0.,-1.,0.));
#31878=DIRECTION('center_axis',(-1.,0.,0.));
#31879=DIRECTION('ref_axis',(0.,-1.,0.));
#31880=DIRECTION('',(-0.38268343236509,0.923879532511287,1.1314261122877E-16));
#31881=DIRECTION('center_axis',(1.,0.,-1.4359375832322E-16));
#31882=DIRECTION('ref_axis',(0.,-1.,0.));
#31883=DIRECTION('center_axis',(1.,0.,-1.4359375832322E-16));
#31884=DIRECTION('ref_axis',(0.,-1.,0.));
#31885=DIRECTION('center_axis',(-1.,0.,0.));
#31886=DIRECTION('ref_axis',(0.,1.,0.));
#31887=DIRECTION('',(-0.707106781186548,-0.707106781186548,-8.65956056235493E-17));
#31888=DIRECTION('center_axis',(-1.,0.,0.));
#31889=DIRECTION('ref_axis',(0.,-1.,0.));
#31890=DIRECTION('center_axis',(-1.,0.,0.));
#31891=DIRECTION('ref_axis',(0.,-1.,0.));
#31892=DIRECTION('center_axis',(1.,0.,0.));
#31893=DIRECTION('ref_axis',(0.,0.,-1.));
#31894=DIRECTION('center_axis',(1.,0.,0.));
#31895=DIRECTION('ref_axis',(0.,0.,-1.));
#31896=DIRECTION('center_axis',(-1.,0.,0.));
#31897=DIRECTION('ref_axis',(0.,0.,1.));
#31898=DIRECTION('center_axis',(-1.,0.,0.));
#31899=DIRECTION('ref_axis',(0.,0.,1.));
#31900=DIRECTION('center_axis',(-1.,0.,0.));
#31901=DIRECTION('ref_axis',(0.,0.,1.));
#31902=DIRECTION('center_axis',(-1.,0.,0.));
#31903=DIRECTION('ref_axis',(0.,0.,1.));
#31904=DIRECTION('center_axis',(-1.,0.,0.));
#31905=DIRECTION('ref_axis',(0.,-1.,0.));
#31906=DIRECTION('',(-0.923879532511287,0.38268343236509,4.6865204053263E-17));
#31907=DIRECTION('center_axis',(1.,0.,0.));
#31908=DIRECTION('ref_axis',(0.,-1.,0.));
#31909=DIRECTION('center_axis',(1.,0.,0.));
#31910=DIRECTION('ref_axis',(0.,-1.,0.));
#31911=DIRECTION('center_axis',(1.,0.,0.));
#31912=DIRECTION('ref_axis',(0.,1.,0.));
#31913=DIRECTION('',(-1.,0.,0.));
#31914=DIRECTION('center_axis',(-1.,0.,0.));
#31915=DIRECTION('ref_axis',(0.,-1.,0.));
#31916=DIRECTION('center_axis',(-1.,0.,0.));
#31917=DIRECTION('ref_axis',(0.,-1.,0.));
#31918=DIRECTION('center_axis',(1.,0.,0.));
#31919=DIRECTION('ref_axis',(0.,-1.,0.));
#31920=DIRECTION('',(-0.923879532511287,-0.38268343236509,-4.6865204053263E-17));
#31921=DIRECTION('center_axis',(1.,0.,0.));
#31922=DIRECTION('ref_axis',(0.,-1.,0.));
#31923=DIRECTION('center_axis',(1.,0.,0.));
#31924=DIRECTION('ref_axis',(0.,-1.,0.));
#31925=DIRECTION('center_axis',(1.,0.,0.));
#31926=DIRECTION('ref_axis',(0.,1.,0.));
#31927=DIRECTION('',(-0.707106781186551,0.707106781186545,8.6595605623549E-17));
#31928=DIRECTION('center_axis',(-1.,0.,-1.4359375832322E-16));
#31929=DIRECTION('ref_axis',(0.,-1.,0.));
#31930=DIRECTION('center_axis',(-1.,0.,-1.4359375832322E-16));
#31931=DIRECTION('ref_axis',(0.,-1.,0.));
#31932=DIRECTION('center_axis',(1.,0.,0.));
#31933=DIRECTION('ref_axis',(0.,-1.,0.));
#31934=DIRECTION('',(-0.38268343236509,-0.923879532511287,-1.1314261122877E-16));
#31935=DIRECTION('center_axis',(1.,0.,0.));
#31936=DIRECTION('ref_axis',(0.,-1.,0.));
#31937=DIRECTION('center_axis',(-1.,0.,0.));
#31938=DIRECTION('ref_axis',(0.,0.,1.));
#31939=DIRECTION('center_axis',(1.,0.,0.));
#31940=DIRECTION('ref_axis',(0.,0.,-1.));
#31941=DIRECTION('center_axis',(1.,0.,0.));
#31942=DIRECTION('ref_axis',(0.,0.,1.));
#31943=DIRECTION('center_axis',(1.,0.,0.));
#31944=DIRECTION('ref_axis',(0.,0.,1.));
#31945=DIRECTION('center_axis',(1.,0.,0.));
#31946=DIRECTION('ref_axis',(0.,0.,1.));
#31947=DIRECTION('center_axis',(1.,0.,0.));
#31948=DIRECTION('ref_axis',(0.,0.,1.));
#31949=DIRECTION('center_axis',(1.,0.,0.));
#31950=DIRECTION('ref_axis',(0.,-1.,0.));
#31951=DIRECTION('center_axis',(-1.,0.,0.));
#31952=DIRECTION('ref_axis',(0.,-1.,0.));
#31953=DIRECTION('center_axis',(-1.,0.,0.));
#31954=DIRECTION('ref_axis',(0.,-1.,0.));
#31955=DIRECTION('',(-0.923879532511288,-0.382683432365086,-4.68652040532625E-17));
#31956=DIRECTION('center_axis',(1.,0.,0.));
#31957=DIRECTION('ref_axis',(0.,-1.,0.));
#31958=DIRECTION('center_axis',(1.,0.,0.));
#31959=DIRECTION('ref_axis',(0.,-1.,0.));
#31960=DIRECTION('center_axis',(1.,0.,0.));
#31961=DIRECTION('ref_axis',(0.,1.,0.));
#31962=DIRECTION('',(-0.707106781186551,0.707106781186544,8.6595605623549E-17));
#31963=DIRECTION('center_axis',(-1.,0.,3.24703122485565E-16));
#31964=DIRECTION('ref_axis',(0.,-1.,0.));
#31965=DIRECTION('center_axis',(-1.,0.,3.24703122485565E-16));
#31966=DIRECTION('ref_axis',(0.,-1.,0.));
#31967=DIRECTION('center_axis',(1.,0.,0.));
#31968=DIRECTION('ref_axis',(0.,1.,0.));
#31969=DIRECTION('',(-1.,0.,0.));
#31970=DIRECTION('center_axis',(1.,0.,0.));
#31971=DIRECTION('ref_axis',(0.,-1.,0.));
#31972=DIRECTION('',(-0.38268343236509,-0.923879532511287,-1.1314261122877E-16));
#31973=DIRECTION('center_axis',(1.,0.,0.));
#31974=DIRECTION('ref_axis',(0.,-1.,0.));
#31975=DIRECTION('center_axis',(-1.,0.,0.));
#31976=DIRECTION('ref_axis',(0.,0.,1.));
#31977=DIRECTION('center_axis',(-1.,0.,0.));
#31978=DIRECTION('ref_axis',(0.,-1.,0.));
#31979=DIRECTION('center_axis',(-1.,0.,0.));
#31980=DIRECTION('ref_axis',(0.,-1.,0.));
#31981=DIRECTION('',(0.707106781186546,-0.707106781186549,8.65956056235495E-17));
#31982=DIRECTION('center_axis',(1.,0.,0.));
#31983=DIRECTION('ref_axis',(0.,-1.,0.));
#31984=DIRECTION('center_axis',(1.,0.,0.));
#31985=DIRECTION('ref_axis',(0.,-1.,0.));
#31986=DIRECTION('center_axis',(1.,0.,0.));
#31987=DIRECTION('ref_axis',(0.,1.,0.));
#31988=DIRECTION('center_axis',(1.,0.,0.));
#31989=DIRECTION('ref_axis',(0.,0.,-1.));
#31990=DIRECTION('',(-1.,0.,0.));
#31991=DIRECTION('center_axis',(-1.,0.,0.));
#31992=DIRECTION('ref_axis',(0.,0.,1.));
#31993=DIRECTION('',(-1.,0.,0.));
#31994=DIRECTION('center_axis',(-1.,0.,0.));
#31995=DIRECTION('ref_axis',(0.,0.,1.));
#31996=DIRECTION('',(-1.,0.,0.));
#31997=DIRECTION('center_axis',(-1.,0.,0.));
#31998=DIRECTION('ref_axis',(0.,0.,1.));
#31999=DIRECTION('',(-1.,0.,0.));
#32000=DIRECTION('center_axis',(-1.,0.,0.));
#32001=DIRECTION('ref_axis',(0.,0.,1.));
#32002=DIRECTION('',(-1.,0.,0.));
#32003=DIRECTION('center_axis',(1.,0.,0.));
#32004=DIRECTION('ref_axis',(0.,1.,0.));
#32005=DIRECTION('center_axis',(1.,0.,0.));
#32006=DIRECTION('ref_axis',(0.,0.,-1.));
#32007=DIRECTION('',(-1.,0.,0.));
#32008=DIRECTION('center_axis',(-1.,0.,0.));
#32009=DIRECTION('ref_axis',(0.,1.,0.));
#32010=DIRECTION('',(-0.707106781186554,-0.707106781186541,-8.65956056235486E-17));
#32011=DIRECTION('center_axis',(1.,0.,0.));
#32012=DIRECTION('ref_axis',(0.,0.,-1.));
#32013=DIRECTION('center_axis',(1.,0.,0.));
#32014=DIRECTION('ref_axis',(0.,0.,-1.));
#32015=DIRECTION('center_axis',(1.,0.,0.));
#32016=DIRECTION('ref_axis',(0.,1.,0.));
#32017=DIRECTION('',(-1.,0.,0.));
#32018=DIRECTION('center_axis',(1.,0.,0.));
#32019=DIRECTION('ref_axis',(0.,0.,-1.));
#32020=DIRECTION('center_axis',(-1.,0.,0.));
#32021=DIRECTION('ref_axis',(0.,0.,1.));
#49688=CARTESIAN_POINT('',(0.,0.,0.));
#49689=CARTESIAN_POINT('Origin',(9.375,0.,26.5));
#49690=CARTESIAN_POINT('',(9.35,1.8,26.5));
#49691=CARTESIAN_POINT('',(9.35,-1.8,26.5));
#49692=CARTESIAN_POINT('Origin',(9.35,0.,26.5));
#49693=CARTESIAN_POINT('Origin',(9.35,0.,26.5));
#49694=CARTESIAN_POINT('',(9.4,1.85,26.5));
#49695=CARTESIAN_POINT('',(9.375,1.825,26.5));
#49696=CARTESIAN_POINT('Origin',(9.4,0.,26.5));
#49697=CARTESIAN_POINT('Origin',(9.4,1.8,26.5));
#49698=CARTESIAN_POINT('',(9.4,-3.445,26.5));
#49699=CARTESIAN_POINT('Origin',(9.4,0.,26.5));
#49700=CARTESIAN_POINT('Origin',(8.6,0.,26.5));
#49701=CARTESIAN_POINT('',(7.8,-1.8,26.5));
#49702=CARTESIAN_POINT('',(8.6,-1.8,26.5));
#49703=CARTESIAN_POINT('Origin',(7.8,0.,26.5));
#49704=CARTESIAN_POINT('Origin',(7.98232233047034,0.,26.5));
#49705=CARTESIAN_POINT('',(8.,6.1,26.5));
#49706=CARTESIAN_POINT('Origin',(8.,0.,26.5));
#49707=CARTESIAN_POINT('',(7.96464466094067,6.18535533905933,26.5));
#49708=CARTESIAN_POINT('',(7.98232233047034,6.14267766952966,26.5));
#49709=CARTESIAN_POINT('',(7.96464466094067,-6.18535533905933,26.5));
#49710=CARTESIAN_POINT('Origin',(7.96464466094067,0.,26.5));
#49711=CARTESIAN_POINT('Origin',(7.96464466094067,0.,26.5));
#49712=CARTESIAN_POINT('Origin',(7.95,0.,26.5));
#49713=CARTESIAN_POINT('',(7.93535533905933,-6.21464466094067,26.5));
#49714=CARTESIAN_POINT('',(7.95,-6.2,26.5));
#49715=CARTESIAN_POINT('',(7.93535533905933,6.21464466094067,26.5));
#49716=CARTESIAN_POINT('Origin',(7.93535533905933,0.,26.5));
#49717=CARTESIAN_POINT('Origin',(7.93535533905933,0.,26.5));
#49718=CARTESIAN_POINT('Origin',(8.,3.495,26.5));
#49719=CARTESIAN_POINT('',(8.,-3.495,26.5));
#49720=CARTESIAN_POINT('Origin',(8.,0.,26.5));
#49721=CARTESIAN_POINT('',(8.,3.53553390593274,29.7055339059327));
#49722=CARTESIAN_POINT('Origin',(8.,3.53553390593274,30.0355339059327));
#49723=CARTESIAN_POINT('',(8.,-3.53553390593274,29.7055339059327));
#49724=CARTESIAN_POINT('Origin',(8.,-3.53553390593274,30.0355339059327));
#49725=CARTESIAN_POINT('',(8.,-3.53553390593274,22.6344660940673));
#49726=CARTESIAN_POINT('Origin',(8.,-3.53553390593274,22.9644660940673));
#49727=CARTESIAN_POINT('',(8.,3.53553390593274,22.6344660940673));
#49728=CARTESIAN_POINT('Origin',(8.,3.53553390593274,22.9644660940673));
#49729=CARTESIAN_POINT('Origin',(7.89267766952966,0.,26.5));
#49730=CARTESIAN_POINT('',(7.85,6.25,26.5));
#49731=CARTESIAN_POINT('',(7.89267766952966,6.23232233047034,26.5));
#49732=CARTESIAN_POINT('',(7.85,-6.25,26.5));
#49733=CARTESIAN_POINT('Origin',(7.85,0.,26.5));
#49734=CARTESIAN_POINT('Origin',(7.85,0.,26.5));
#49735=CARTESIAN_POINT('Origin',(7.4,0.,26.5));
#49736=CARTESIAN_POINT('',(6.95,-6.25,26.5));
#49737=CARTESIAN_POINT('',(7.4,-6.25,26.5));
#49738=CARTESIAN_POINT('',(6.95,6.25,26.5));
#49739=CARTESIAN_POINT('Origin',(6.95,0.,26.5));
#49740=CARTESIAN_POINT('Origin',(6.95,0.,26.5));
#49741=CARTESIAN_POINT('Origin',(6.90732233047034,0.,26.5));
#49742=CARTESIAN_POINT('',(6.86464466094067,6.21464466094067,26.5));
#49743=CARTESIAN_POINT('',(6.90732233047034,6.23232233047034,26.5));
#49744=CARTESIAN_POINT('',(6.86464466094067,-6.21464466094067,26.5));
#49745=CARTESIAN_POINT('Origin',(6.86464466094067,0.,26.5));
#49746=CARTESIAN_POINT('Origin',(6.86464466094067,0.,26.5));
#49747=CARTESIAN_POINT('Origin',(6.85,0.,26.5));
#49748=CARTESIAN_POINT('',(6.83535533905933,-6.18535533905933,26.5));
#49749=CARTESIAN_POINT('',(6.85,-6.2,26.5));
#49750=CARTESIAN_POINT('',(6.83535533905933,6.18535533905933,26.5));
#49751=CARTESIAN_POINT('Origin',(6.83535533905933,0.,26.5));
#49752=CARTESIAN_POINT('Origin',(6.83535533905933,0.,26.5));
#49753=CARTESIAN_POINT('Origin',(6.81767766952966,0.,26.5));
#49754=CARTESIAN_POINT('',(6.8,6.1,26.5));
#49755=CARTESIAN_POINT('',(6.81767766952966,6.14267766952966,26.5));
#49756=CARTESIAN_POINT('Origin',(6.8,0.,26.5));
#49757=CARTESIAN_POINT('Origin',(6.8,6.15,26.5));
#49758=CARTESIAN_POINT('',(6.8,-2.8,26.5));
#49759=CARTESIAN_POINT('Origin',(6.8,0.,26.5));
#49760=CARTESIAN_POINT('',(6.8,3.53553390593274,29.7055339059327));
#49761=CARTESIAN_POINT('Origin',(6.8,3.53553390593274,30.0355339059327));
#49762=CARTESIAN_POINT('',(6.8,-3.53553390593274,29.7055339059327));
#49763=CARTESIAN_POINT('Origin',(6.8,-3.53553390593274,30.0355339059327));
#49764=CARTESIAN_POINT('',(6.8,-3.53553390593274,22.6344660940673));
#49765=CARTESIAN_POINT('Origin',(6.8,-3.53553390593274,22.9644660940673));
#49766=CARTESIAN_POINT('',(6.8,3.53553390593274,22.6344660940673));
#49767=CARTESIAN_POINT('Origin',(6.8,3.53553390593274,22.9644660940673));
#49768=CARTESIAN_POINT('Origin',(5.15732233047034,0.,26.5));
#49769=CARTESIAN_POINT('',(5.2,2.8,26.5));
#49770=CARTESIAN_POINT('',(5.2,-2.8,26.5));
#49771=CARTESIAN_POINT('Origin',(5.2,0.,26.5));
#49772=CARTESIAN_POINT('Origin',(5.2,0.,26.5));
#49773=CARTESIAN_POINT('',(5.11464466094067,2.76464466094067,26.5));
#49774=CARTESIAN_POINT('',(5.15732233047034,2.78232233047034,26.5));
#49775=CARTESIAN_POINT('',(5.11464466094067,-2.76464466094067,26.5));
#49776=CARTESIAN_POINT('Origin',(5.11464466094067,0.,26.5));
#49777=CARTESIAN_POINT('Origin',(5.11464466094067,0.,26.5));
#49778=CARTESIAN_POINT('Origin',(5.1,0.,26.5));
#49779=CARTESIAN_POINT('',(5.08535533905933,-2.73535533905933,26.5));
#49780=CARTESIAN_POINT('',(5.1,-2.75,26.5));
#49781=CARTESIAN_POINT('',(5.08535533905933,2.73535533905933,26.5));
#49782=CARTESIAN_POINT('Origin',(5.08535533905933,0.,26.5));
#49783=CARTESIAN_POINT('Origin',(5.08535533905933,0.,26.5));
#49784=CARTESIAN_POINT('Origin',(5.975,0.,26.5));
#49785=CARTESIAN_POINT('',(5.975,-2.8,26.5));
#49786=CARTESIAN_POINT('Origin',(5.06767766952966,0.,26.5));
#49787=CARTESIAN_POINT('',(5.05,2.65,26.5));
#49788=CARTESIAN_POINT('',(5.06767766952966,2.69267766952966,26.5));
#49789=CARTESIAN_POINT('Origin',(5.05,0.,26.5));
#49790=CARTESIAN_POINT('Origin',(5.05,2.7,26.5));
#49791=CARTESIAN_POINT('',(5.05,1.85,26.5));
#49792=CARTESIAN_POINT('Origin',(5.05,0.,26.5));
#49793=CARTESIAN_POINT('Origin',(5.075,0.,26.5));
#49794=CARTESIAN_POINT('',(5.1,1.8,26.5));
#49795=CARTESIAN_POINT('',(5.075,1.825,26.5));
#49796=CARTESIAN_POINT('',(5.1,-1.8,26.5));
#49797=CARTESIAN_POINT('Origin',(5.1,0.,26.5));
#49798=CARTESIAN_POINT('Origin',(5.1,0.,26.5));
#49799=CARTESIAN_POINT('Origin',(5.525,0.,26.5));
#49800=CARTESIAN_POINT('',(6.,-1.8,26.5));
#49801=CARTESIAN_POINT('Origin',(6.,0.,26.5));
#49802=CARTESIAN_POINT('',(5.525,-1.8,26.5));
#49803=CARTESIAN_POINT('Origin',(7.41,3.53553390593274,22.9644660940673));
#49804=CARTESIAN_POINT('',(7.41,3.53553390593274,22.6344660940673));
#49805=CARTESIAN_POINT('Origin',(7.41,-3.53553390593274,22.9644660940673));
#49806=CARTESIAN_POINT('',(7.41,-3.53553390593274,22.6344660940673));
#49807=CARTESIAN_POINT('Origin',(7.41,-3.53553390593274,30.0355339059327));
#49808=CARTESIAN_POINT('',(7.41,-3.53553390593274,29.7055339059327));
#49809=CARTESIAN_POINT('Origin',(7.41,3.53553390593274,30.0355339059327));
#49810=CARTESIAN_POINT('',(7.41,3.53553390593274,29.7055339059327));
#49811=CARTESIAN_POINT('Origin',(8.675,0.,26.5));
#49812=CARTESIAN_POINT('',(9.35,-3.495,26.5));
#49813=CARTESIAN_POINT('Origin',(9.35,0.,26.5));
#49814=CARTESIAN_POINT('',(8.675,-3.495,26.5));
#49815=CARTESIAN_POINT('Origin',(9.375,0.,26.5));
#49816=CARTESIAN_POINT('',(9.375,-3.47,26.5));
#49817=CARTESIAN_POINT('Origin',(7.8,1.05,26.5));
#49818=CARTESIAN_POINT('',(7.8,-1.05,26.5));
#49819=CARTESIAN_POINT('Origin',(7.8,0.,26.5));
#49820=CARTESIAN_POINT('Origin',(6.9,0.,26.5));
#49821=CARTESIAN_POINT('',(6.,-1.05,26.5));
#49822=CARTESIAN_POINT('',(6.9,-1.05,26.5));
#49823=CARTESIAN_POINT('Origin',(6.,0.,26.5));
#49824=CARTESIAN_POINT('Origin',(6.,1.8,26.5));
#76624=UNCERTAINTY_MEASURE_WITH_UNIT(LENGTH_MEASURE(0.001),#76661,
'DISTANCE_ACCURACY_VALUE',
'Maximum model space distance between geometric entities at asserted c
onnectivities');
#76638=UNCERTAINTY_MEASURE_WITH_UNIT(LENGTH_MEASURE(0.001),#76661,
'DISTANCE_ACCURACY_VALUE',
'Maximum model space distance between geometric entities at asserted c
onnectivities');
#76646=(
GEOMETRIC_REPRESENTATION_CONTEXT(3)
GLOBAL_UNCERTAINTY_ASSIGNED_CONTEXT((#76624))
GLOBAL_UNIT_ASSIGNED_CONTEXT((#76661,#76663,#76664))
REPRESENTATION_CONTEXT('','3D')
);
#76660=(
GEOMETRIC_REPRESENTATION_CONTEXT(3)
GLOBAL_UNCERTAINTY_ASSIGNED_CONTEXT((#76638))
GLOBAL_UNIT_ASSIGNED_CONTEXT((#76661,#76663,#76664))
REPRESENTATION_CONTEXT('','3D')
);
#76661=(
LENGTH_UNIT()
NAMED_UNIT(*)
SI_UNIT(.CENTI.,.METRE.)
);
#76663=(
NAMED_UNIT(*)
PLANE_ANGLE_UNIT()
SI_UNIT($,.RADIAN.)
);
#76664=(
NAMED_UNIT(*)
SI_UNIT($,.STERADIAN.)
SOLID_ANGLE_UNIT()
);
#76672=SHAPE_DEFINITION_REPRESENTATION(#76693,#76742);
#76693=PRODUCT_DEFINITION_SHAPE('',$,#76764);
#76742=SHAPE_REPRESENTATION('',(#27753),#76646);
#76756=PRODUCT_DEFINITION_CONTEXT('part definition',#76821,'design');
#76764=PRODUCT_DEFINITION('2026-10-26-11-12-49-269',
'07_Rear_Bearing_Cap_D125',#76785,#76756);
#76785=PRODUCT_DEFINITION_FORMATION('',$,#76830);
#76821=APPLICATION_CONTEXT(
'Core Data for Automotive Mechanical Design Process');
#76822=PRODUCT_CONTEXT('part definition',#76821,'mechanical');
#76830=PRODUCT('2026-10-26-11-12-49-269','07_Rear_Bearing_Cap_D125',$,(#76822));
#76900=COLOUR_RGB('Grey',0.48,0.52,0.57);
#76901=FILL_AREA_STYLE_COLOUR('',#76900);
#76902=FILL_AREA_STYLE('',(#76901));
#76903=SURFACE_STYLE_FILL_AREA(#76902);
#76904=SURFACE_SIDE_STYLE('',(#76903));
#76905=SURFACE_STYLE_USAGE(.BOTH.,#76904);
#76906=PRESENTATION_STYLE_ASSIGNMENT((#76905));
ENDSEC;
END-ISO-10303-21;
